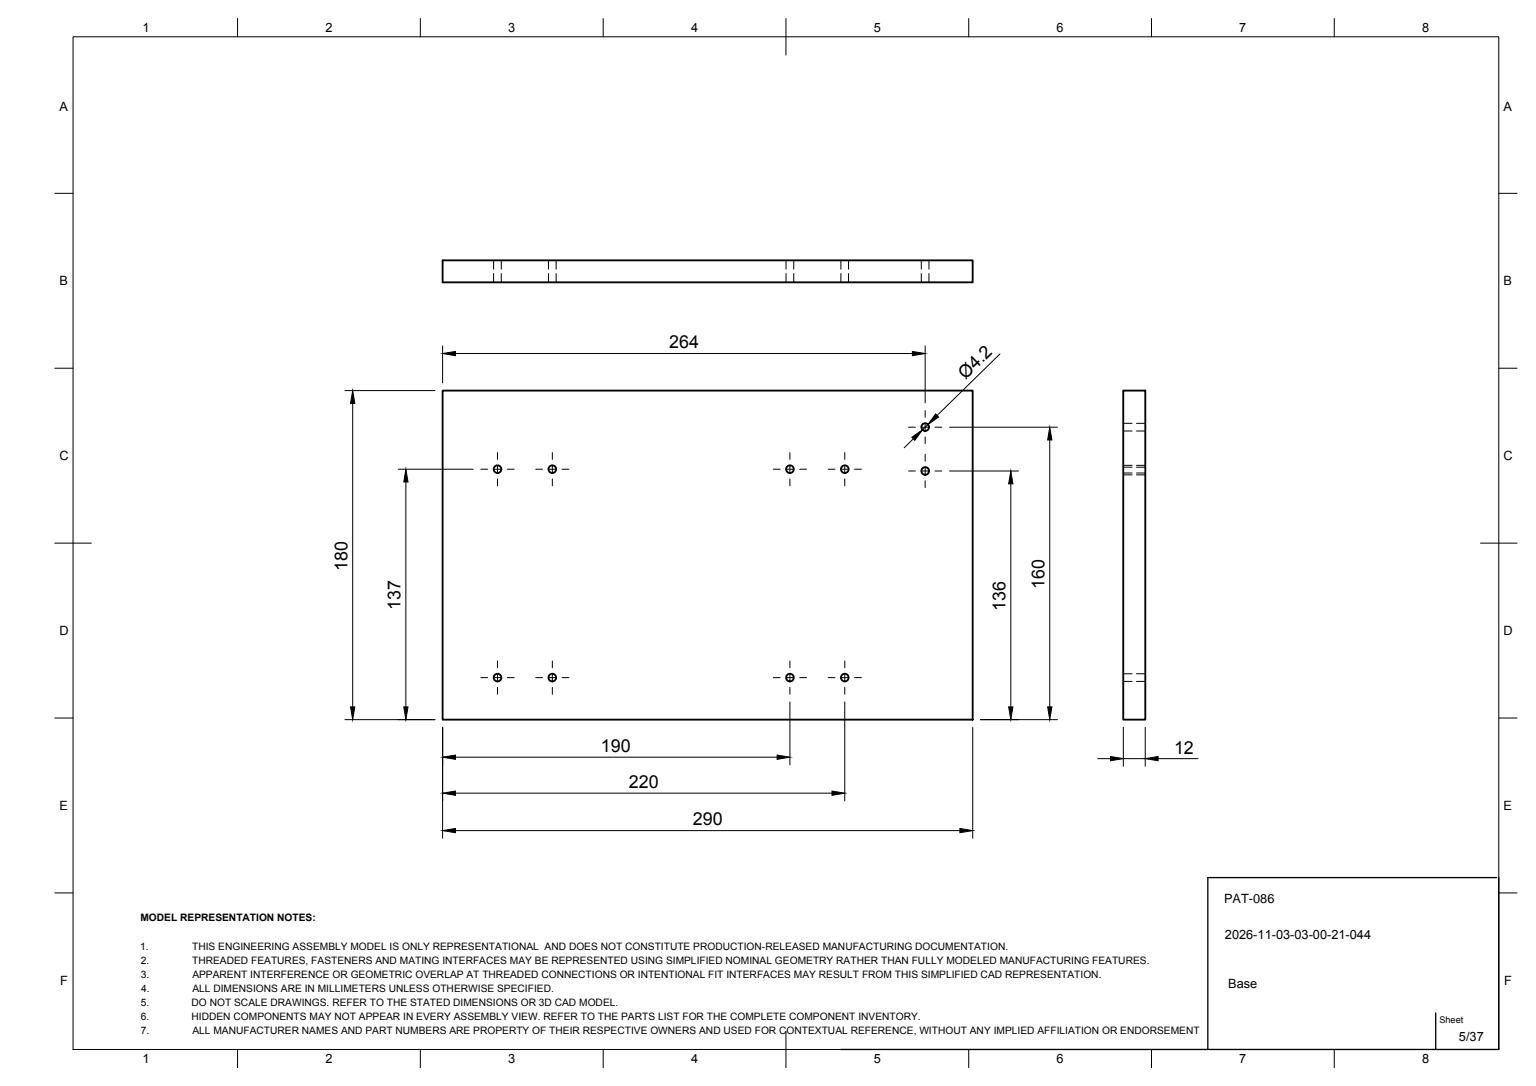
ISO-10303-21;
HEADER;
/* Generated by software containing ST-Developer
 * from STEP Tools, Inc. (www.steptools.com) 
 */

FILE_DESCRIPTION(
/* description */ ('Ratchet and pawl hand winch drum'),
/* implementation_level */ '2;1');

FILE_NAME(
/* name */ 'Base.step',
/* time_stamp */ '2026-10-27T12:42:58-07:00',
/* author */ (''),
/* organization */ (''),
/* preprocessor_version */ 'ST-DEVELOPER v20.2',
/* originating_system */ 'Autodesk Translation Framework v15.17.0.0',
/* authorisation */ '');

FILE_SCHEMA (('AUTOMOTIVE_DESIGN { 1 0 10303 214 3 1 1 }'));
ENDSEC;

DATA;
#10=MECHANICAL_DESIGN_GEOMETRIC_PRESENTATION_REPRESENTATION('',(#389),#11801);
#321=SHAPE_REPRESENTATION_RELATIONSHIP('SRR','None',#11947,#355);
#355=ADVANCED_BREP_SHAPE_REPRESENTATION('',(#424),#11764);
#389=STYLED_ITEM('',(#12192),#424);
#424=MANIFOLD_SOLID_BREP('Body1',#6266);
#456=FACE_BOUND('',#1211,.T.);
#457=FACE_BOUND('',#1212,.T.);
#458=FACE_BOUND('',#1213,.T.);
#459=FACE_BOUND('',#1214,.T.);
#460=FACE_BOUND('',#1215,.T.);
#461=FACE_BOUND('',#1216,.T.);
#462=FACE_BOUND('',#1217,.T.);
#463=FACE_BOUND('',#1218,.T.);
#464=FACE_BOUND('',#1219,.T.);
#465=FACE_BOUND('',#1220,.T.);
#466=FACE_BOUND('',#1222,.T.);
#467=FACE_BOUND('',#1223,.T.);
#468=FACE_BOUND('',#1224,.T.);
#469=FACE_BOUND('',#1225,.T.);
#470=FACE_BOUND('',#1226,.T.);
#471=FACE_BOUND('',#1227,.T.);
#472=FACE_BOUND('',#1228,.T.);
#473=FACE_BOUND('',#1229,.T.);
#474=FACE_BOUND('',#1230,.T.);
#475=FACE_BOUND('',#1231,.T.);
#601=PLANE('',#6712);
#602=PLANE('',#6713);
#603=PLANE('',#6714);
#604=PLANE('',#6715);
#605=PLANE('',#6716);
#606=PLANE('',#6717);
#840=FACE_OUTER_BOUND('',#1196,.T.);
#841=FACE_OUTER_BOUND('',#1197,.T.);
#842=FACE_OUTER_BOUND('',#1198,.T.);
#843=FACE_OUTER_BOUND('',#1199,.T.);
#844=FACE_OUTER_BOUND('',#1200,.T.);
#845=FACE_OUTER_BOUND('',#1201,.T.);
#846=FACE_OUTER_BOUND('',#1202,.T.);
#847=FACE_OUTER_BOUND('',#1203,.T.);
#848=FACE_OUTER_BOUND('',#1204,.T.);
#849=FACE_OUTER_BOUND('',#1205,.T.);
#850=FACE_OUTER_BOUND('',#1206,.T.);
#851=FACE_OUTER_BOUND('',#1207,.T.);
#852=FACE_OUTER_BOUND('',#1208,.T.);
#853=FACE_OUTER_BOUND('',#1209,.T.);
#854=FACE_OUTER_BOUND('',#1210,.T.);
#855=FACE_OUTER_BOUND('',#1221,.T.);
#1196=EDGE_LOOP('',(#4247,#4248,#4249,#4250));
#1197=EDGE_LOOP('',(#4251,#4252,#4253,#4254));
#1198=EDGE_LOOP('',(#4255,#4256,#4257,#4258));
#1199=EDGE_LOOP('',(#4259,#4260,#4261,#4262));
#1200=EDGE_LOOP('',(#4263,#4264,#4265,#4266));
#1201=EDGE_LOOP('',(#4267,#4268,#4269,#4270));
#1202=EDGE_LOOP('',(#4271,#4272,#4273,#4274));
#1203=EDGE_LOOP('',(#4275,#4276,#4277,#4278));
#1204=EDGE_LOOP('',(#4279,#4280,#4281,#4282));
#1205=EDGE_LOOP('',(#4283,#4284,#4285,#4286));
#1206=EDGE_LOOP('',(#4287,#4288,#4289,#4290));
#1207=EDGE_LOOP('',(#4291,#4292,#4293,#4294));
#1208=EDGE_LOOP('',(#4295,#4296,#4297,#4298));
#1209=EDGE_LOOP('',(#4299,#4300,#4301,#4302));
#1210=EDGE_LOOP('',(#4303,#4304,#4305,#4306));
#1211=EDGE_LOOP('',(#4307));
#1212=EDGE_LOOP('',(#4308));
#1213=EDGE_LOOP('',(#4309));
#1214=EDGE_LOOP('',(#4310));
#1215=EDGE_LOOP('',(#4311));
#1216=EDGE_LOOP('',(#4312));
#1217=EDGE_LOOP('',(#4313));
#1218=EDGE_LOOP('',(#4314));
#1219=EDGE_LOOP('',(#4315));
#1220=EDGE_LOOP('',(#4316));
#1221=EDGE_LOOP('',(#4317,#4318,#4319,#4320));
#1222=EDGE_LOOP('',(#4321));
#1223=EDGE_LOOP('',(#4322));
#1224=EDGE_LOOP('',(#4323));
#1225=EDGE_LOOP('',(#4324));
#1226=EDGE_LOOP('',(#4325));
#1227=EDGE_LOOP('',(#4326));
#1228=EDGE_LOOP('',(#4327));
#1229=EDGE_LOOP('',(#4328));
#1230=EDGE_LOOP('',(#4329));
#1231=EDGE_LOOP('',(#4330));
#1697=LINE('',#9234,#2208);
#1698=LINE('',#9240,#2209);
#1699=LINE('',#9246,#2210);
#1700=LINE('',#9252,#2211);
#1701=LINE('',#9258,#2212);
#1702=LINE('',#9264,#2213);
#1703=LINE('',#9270,#2214);
#1704=LINE('',#9276,#2215);
#1705=LINE('',#9282,#2216);
#1706=LINE('',#9288,#2217);
#1707=LINE('',#9293,#2218);
#1708=LINE('',#9295,#2219);
#1709=LINE('',#9297,#2220);
#1710=LINE('',#9298,#2221);
#1711=LINE('',#9301,#2222);
#1712=LINE('',#9303,#2223);
#1713=LINE('',#9304,#2224);
#1714=LINE('',#9307,#2225);
#1715=LINE('',#9309,#2226);
#1716=LINE('',#9310,#2227);
#1717=LINE('',#9312,#2228);
#1718=LINE('',#9313,#2229);
#2208=VECTOR('',#7368,0.210000000000001);
#2209=VECTOR('',#7375,0.21);
#2210=VECTOR('',#7382,0.21);
#2211=VECTOR('',#7389,0.21);
#2212=VECTOR('',#7396,0.21);
#2213=VECTOR('',#7403,0.21);
#2214=VECTOR('',#7410,0.21);
#2215=VECTOR('',#7417,0.21);
#2216=VECTOR('',#7424,0.21);
#2217=VECTOR('',#7431,0.21);
#2218=VECTOR('',#7436,1.);
#2219=VECTOR('',#7437,1.);
#2220=VECTOR('',#7438,1.);
#2221=VECTOR('',#7439,1.);
#2222=VECTOR('',#7442,1.);
#2223=VECTOR('',#7443,1.);
#2224=VECTOR('',#7444,1.);
#2225=VECTOR('',#7447,1.);
#2226=VECTOR('',#7448,1.);
#2227=VECTOR('',#7449,1.);
#2228=VECTOR('',#7452,1.);
#2229=VECTOR('',#7453,1.);
#2719=CIRCLE('',#6683,0.210000000000001);
#2720=CIRCLE('',#6684,0.210000000000001);
#2721=CIRCLE('',#6686,0.21);
#2722=CIRCLE('',#6687,0.21);
#2723=CIRCLE('',#6689,0.21);
#2724=CIRCLE('',#6690,0.21);
#2725=CIRCLE('',#6692,0.21);
#2726=CIRCLE('',#6693,0.21);
#2727=CIRCLE('',#6695,0.21);
#2728=CIRCLE('',#6696,0.21);
#2729=CIRCLE('',#6698,0.21);
#2730=CIRCLE('',#6699,0.21);
#2731=CIRCLE('',#6701,0.21);
#2732=CIRCLE('',#6702,0.21);
#2733=CIRCLE('',#6704,0.21);
#2734=CIRCLE('',#6705,0.21);
#2735=CIRCLE('',#6707,0.21);
#2736=CIRCLE('',#6708,0.21);
#2737=CIRCLE('',#6710,0.21);
#2738=CIRCLE('',#6711,0.21);
#2942=VERTEX_POINT('',#9231);
#2943=VERTEX_POINT('',#9233);
#2944=VERTEX_POINT('',#9237);
#2945=VERTEX_POINT('',#9239);
#2946=VERTEX_POINT('',#9243);
#2947=VERTEX_POINT('',#9245);
#2948=VERTEX_POINT('',#9249);
#2949=VERTEX_POINT('',#9251);
#2950=VERTEX_POINT('',#9255);
#2951=VERTEX_POINT('',#9257);
#2952=VERTEX_POINT('',#9261);
#2953=VERTEX_POINT('',#9263);
#2954=VERTEX_POINT('',#9267);
#2955=VERTEX_POINT('',#9269);
#2956=VERTEX_POINT('',#9273);
#2957=VERTEX_POINT('',#9275);
#2958=VERTEX_POINT('',#9279);
#2959=VERTEX_POINT('',#9281);
#2960=VERTEX_POINT('',#9285);
#2961=VERTEX_POINT('',#9287);
#2962=VERTEX_POINT('',#9291);
#2963=VERTEX_POINT('',#9292);
#2964=VERTEX_POINT('',#9294);
#2965=VERTEX_POINT('',#9296);
#2966=VERTEX_POINT('',#9300);
#2967=VERTEX_POINT('',#9302);
#2968=VERTEX_POINT('',#9306);
#2969=VERTEX_POINT('',#9308);
#3467=EDGE_CURVE('',#2942,#2942,#2719,.T.);
#3468=EDGE_CURVE('',#2942,#2943,#1697,.T.);
#3469=EDGE_CURVE('',#2943,#2943,#2720,.T.);
#3470=EDGE_CURVE('',#2944,#2944,#2721,.T.);
#3471=EDGE_CURVE('',#2944,#2945,#1698,.T.);
#3472=EDGE_CURVE('',#2945,#2945,#2722,.T.);
#3473=EDGE_CURVE('',#2946,#2946,#2723,.T.);
#3474=EDGE_CURVE('',#2946,#2947,#1699,.T.);
#3475=EDGE_CURVE('',#2947,#2947,#2724,.T.);
#3476=EDGE_CURVE('',#2948,#2948,#2725,.T.);
#3477=EDGE_CURVE('',#2948,#2949,#1700,.T.);
#3478=EDGE_CURVE('',#2949,#2949,#2726,.T.);
#3479=EDGE_CURVE('',#2950,#2950,#2727,.T.);
#3480=EDGE_CURVE('',#2950,#2951,#1701,.T.);
#3481=EDGE_CURVE('',#2951,#2951,#2728,.T.);
#3482=EDGE_CURVE('',#2952,#2952,#2729,.T.);
#3483=EDGE_CURVE('',#2952,#2953,#1702,.T.);
#3484=EDGE_CURVE('',#2953,#2953,#2730,.T.);
#3485=EDGE_CURVE('',#2954,#2954,#2731,.T.);
#3486=EDGE_CURVE('',#2954,#2955,#1703,.T.);
#3487=EDGE_CURVE('',#2955,#2955,#2732,.T.);
#3488=EDGE_CURVE('',#2956,#2956,#2733,.T.);
#3489=EDGE_CURVE('',#2956,#2957,#1704,.T.);
#3490=EDGE_CURVE('',#2957,#2957,#2734,.T.);
#3491=EDGE_CURVE('',#2958,#2958,#2735,.T.);
#3492=EDGE_CURVE('',#2958,#2959,#1705,.T.);
#3493=EDGE_CURVE('',#2959,#2959,#2736,.T.);
#3494=EDGE_CURVE('',#2960,#2960,#2737,.T.);
#3495=EDGE_CURVE('',#2960,#2961,#1706,.T.);
#3496=EDGE_CURVE('',#2961,#2961,#2738,.T.);
#3497=EDGE_CURVE('',#2962,#2963,#1707,.T.);
#3498=EDGE_CURVE('',#2963,#2964,#1708,.T.);
#3499=EDGE_CURVE('',#2965,#2964,#1709,.T.);
#3500=EDGE_CURVE('',#2962,#2965,#1710,.T.);
#3501=EDGE_CURVE('',#2966,#2962,#1711,.T.);
#3502=EDGE_CURVE('',#2967,#2965,#1712,.T.);
#3503=EDGE_CURVE('',#2966,#2967,#1713,.T.);
#3504=EDGE_CURVE('',#2968,#2966,#1714,.T.);
#3505=EDGE_CURVE('',#2969,#2967,#1715,.T.);
#3506=EDGE_CURVE('',#2968,#2969,#1716,.T.);
#3507=EDGE_CURVE('',#2963,#2968,#1717,.T.);
#3508=EDGE_CURVE('',#2964,#2969,#1718,.T.);
#4247=ORIENTED_EDGE('',*,*,#3467,.F.);
#4248=ORIENTED_EDGE('',*,*,#3468,.T.);
#4249=ORIENTED_EDGE('',*,*,#3469,.F.);
#4250=ORIENTED_EDGE('',*,*,#3468,.F.);
#4251=ORIENTED_EDGE('',*,*,#3470,.F.);
#4252=ORIENTED_EDGE('',*,*,#3471,.T.);
#4253=ORIENTED_EDGE('',*,*,#3472,.F.);
#4254=ORIENTED_EDGE('',*,*,#3471,.F.);
#4255=ORIENTED_EDGE('',*,*,#3473,.F.);
#4256=ORIENTED_EDGE('',*,*,#3474,.T.);
#4257=ORIENTED_EDGE('',*,*,#3475,.F.);
#4258=ORIENTED_EDGE('',*,*,#3474,.F.);
#4259=ORIENTED_EDGE('',*,*,#3476,.F.);
#4260=ORIENTED_EDGE('',*,*,#3477,.T.);
#4261=ORIENTED_EDGE('',*,*,#3478,.F.);
#4262=ORIENTED_EDGE('',*,*,#3477,.F.);
#4263=ORIENTED_EDGE('',*,*,#3479,.F.);
#4264=ORIENTED_EDGE('',*,*,#3480,.T.);
#4265=ORIENTED_EDGE('',*,*,#3481,.F.);
#4266=ORIENTED_EDGE('',*,*,#3480,.F.);
#4267=ORIENTED_EDGE('',*,*,#3482,.F.);
#4268=ORIENTED_EDGE('',*,*,#3483,.T.);
#4269=ORIENTED_EDGE('',*,*,#3484,.F.);
#4270=ORIENTED_EDGE('',*,*,#3483,.F.);
#4271=ORIENTED_EDGE('',*,*,#3485,.F.);
#4272=ORIENTED_EDGE('',*,*,#3486,.T.);
#4273=ORIENTED_EDGE('',*,*,#3487,.F.);
#4274=ORIENTED_EDGE('',*,*,#3486,.F.);
#4275=ORIENTED_EDGE('',*,*,#3488,.F.);
#4276=ORIENTED_EDGE('',*,*,#3489,.T.);
#4277=ORIENTED_EDGE('',*,*,#3490,.F.);
#4278=ORIENTED_EDGE('',*,*,#3489,.F.);
#4279=ORIENTED_EDGE('',*,*,#3491,.F.);
#4280=ORIENTED_EDGE('',*,*,#3492,.T.);
#4281=ORIENTED_EDGE('',*,*,#3493,.F.);
#4282=ORIENTED_EDGE('',*,*,#3492,.F.);
#4283=ORIENTED_EDGE('',*,*,#3494,.F.);
#4284=ORIENTED_EDGE('',*,*,#3495,.T.);
#4285=ORIENTED_EDGE('',*,*,#3496,.F.);
#4286=ORIENTED_EDGE('',*,*,#3495,.F.);
#4287=ORIENTED_EDGE('',*,*,#3497,.T.);
#4288=ORIENTED_EDGE('',*,*,#3498,.T.);
#4289=ORIENTED_EDGE('',*,*,#3499,.F.);
#4290=ORIENTED_EDGE('',*,*,#3500,.F.);
#4291=ORIENTED_EDGE('',*,*,#3501,.T.);
#4292=ORIENTED_EDGE('',*,*,#3500,.T.);
#4293=ORIENTED_EDGE('',*,*,#3502,.F.);
#4294=ORIENTED_EDGE('',*,*,#3503,.F.);
#4295=ORIENTED_EDGE('',*,*,#3504,.T.);
#4296=ORIENTED_EDGE('',*,*,#3503,.T.);
#4297=ORIENTED_EDGE('',*,*,#3505,.F.);
#4298=ORIENTED_EDGE('',*,*,#3506,.F.);
#4299=ORIENTED_EDGE('',*,*,#3507,.T.);
#4300=ORIENTED_EDGE('',*,*,#3506,.T.);
#4301=ORIENTED_EDGE('',*,*,#3508,.F.);
#4302=ORIENTED_EDGE('',*,*,#3498,.F.);
#4303=ORIENTED_EDGE('',*,*,#3508,.T.);
#4304=ORIENTED_EDGE('',*,*,#3505,.T.);
#4305=ORIENTED_EDGE('',*,*,#3502,.T.);
#4306=ORIENTED_EDGE('',*,*,#3499,.T.);
#4307=ORIENTED_EDGE('',*,*,#3472,.T.);
#4308=ORIENTED_EDGE('',*,*,#3496,.T.);
#4309=ORIENTED_EDGE('',*,*,#3493,.T.);
#4310=ORIENTED_EDGE('',*,*,#3490,.T.);
#4311=ORIENTED_EDGE('',*,*,#3487,.T.);
#4312=ORIENTED_EDGE('',*,*,#3484,.T.);
#4313=ORIENTED_EDGE('',*,*,#3481,.T.);
#4314=ORIENTED_EDGE('',*,*,#3478,.T.);
#4315=ORIENTED_EDGE('',*,*,#3475,.T.);
#4316=ORIENTED_EDGE('',*,*,#3469,.T.);
#4317=ORIENTED_EDGE('',*,*,#3507,.F.);
#4318=ORIENTED_EDGE('',*,*,#3497,.F.);
#4319=ORIENTED_EDGE('',*,*,#3501,.F.);
#4320=ORIENTED_EDGE('',*,*,#3504,.F.);
#4321=ORIENTED_EDGE('',*,*,#3470,.T.);
#4322=ORIENTED_EDGE('',*,*,#3494,.T.);
#4323=ORIENTED_EDGE('',*,*,#3491,.T.);
#4324=ORIENTED_EDGE('',*,*,#3488,.T.);
#4325=ORIENTED_EDGE('',*,*,#3485,.T.);
#4326=ORIENTED_EDGE('',*,*,#3482,.T.);
#4327=ORIENTED_EDGE('',*,*,#3479,.T.);
#4328=ORIENTED_EDGE('',*,*,#3476,.T.);
#4329=ORIENTED_EDGE('',*,*,#3473,.T.);
#4330=ORIENTED_EDGE('',*,*,#3467,.T.);
#5807=CYLINDRICAL_SURFACE('',#6682,0.210000000000001);
#5808=CYLINDRICAL_SURFACE('',#6685,0.21);
#5809=CYLINDRICAL_SURFACE('',#6688,0.21);
#5810=CYLINDRICAL_SURFACE('',#6691,0.21);
#5811=CYLINDRICAL_SURFACE('',#6694,0.21);
#5812=CYLINDRICAL_SURFACE('',#6697,0.21);
#5813=CYLINDRICAL_SURFACE('',#6700,0.21);
#5814=CYLINDRICAL_SURFACE('',#6703,0.21);
#5815=CYLINDRICAL_SURFACE('',#6706,0.21);
#5816=CYLINDRICAL_SURFACE('',#6709,0.21);
#5910=ADVANCED_FACE('',(#840),#5807,.F.);
#5911=ADVANCED_FACE('',(#841),#5808,.F.);
#5912=ADVANCED_FACE('',(#842),#5809,.F.);
#5913=ADVANCED_FACE('',(#843),#5810,.F.);
#5914=ADVANCED_FACE('',(#844),#5811,.F.);
#5915=ADVANCED_FACE('',(#845),#5812,.F.);
#5916=ADVANCED_FACE('',(#846),#5813,.F.);
#5917=ADVANCED_FACE('',(#847),#5814,.F.);
#5918=ADVANCED_FACE('',(#848),#5815,.F.);
#5919=ADVANCED_FACE('',(#849),#5816,.F.);
#5920=ADVANCED_FACE('',(#850),#601,.T.);
#5921=ADVANCED_FACE('',(#851),#602,.T.);
#5922=ADVANCED_FACE('',(#852),#603,.T.);
#5923=ADVANCED_FACE('',(#853),#604,.T.);
#5924=ADVANCED_FACE('',(#854,#456,#457,#458,#459,#460,#461,#462,#463,#464,
#465),#605,.T.);
#5925=ADVANCED_FACE('',(#855,#466,#467,#468,#469,#470,#471,#472,#473,#474,
#475),#606,.F.);
#6266=CLOSED_SHELL('',(#5910,#5911,#5912,#5913,#5914,#5915,#5916,#5917,
#5918,#5919,#5920,#5921,#5922,#5923,#5924,#5925));
#6681=AXIS2_PLACEMENT_3D('',#9229,#7362,#7363);
#6682=AXIS2_PLACEMENT_3D('',#9230,#7364,#7365);
#6683=AXIS2_PLACEMENT_3D('',#9232,#7366,#7367);
#6684=AXIS2_PLACEMENT_3D('',#9235,#7369,#7370);
#6685=AXIS2_PLACEMENT_3D('',#9236,#7371,#7372);
#6686=AXIS2_PLACEMENT_3D('',#9238,#7373,#7374);
#6687=AXIS2_PLACEMENT_3D('',#9241,#7376,#7377);
#6688=AXIS2_PLACEMENT_3D('',#9242,#7378,#7379);
#6689=AXIS2_PLACEMENT_3D('',#9244,#7380,#7381);
#6690=AXIS2_PLACEMENT_3D('',#9247,#7383,#7384);
#6691=AXIS2_PLACEMENT_3D('',#9248,#7385,#7386);
#6692=AXIS2_PLACEMENT_3D('',#9250,#7387,#7388);
#6693=AXIS2_PLACEMENT_3D('',#9253,#7390,#7391);
#6694=AXIS2_PLACEMENT_3D('',#9254,#7392,#7393);
#6695=AXIS2_PLACEMENT_3D('',#9256,#7394,#7395);
#6696=AXIS2_PLACEMENT_3D('',#9259,#7397,#7398);
#6697=AXIS2_PLACEMENT_3D('',#9260,#7399,#7400);
#6698=AXIS2_PLACEMENT_3D('',#9262,#7401,#7402);
#6699=AXIS2_PLACEMENT_3D('',#9265,#7404,#7405);
#6700=AXIS2_PLACEMENT_3D('',#9266,#7406,#7407);
#6701=AXIS2_PLACEMENT_3D('',#9268,#7408,#7409);
#6702=AXIS2_PLACEMENT_3D('',#9271,#7411,#7412);
#6703=AXIS2_PLACEMENT_3D('',#9272,#7413,#7414);
#6704=AXIS2_PLACEMENT_3D('',#9274,#7415,#7416);
#6705=AXIS2_PLACEMENT_3D('',#9277,#7418,#7419);
#6706=AXIS2_PLACEMENT_3D('',#9278,#7420,#7421);
#6707=AXIS2_PLACEMENT_3D('',#9280,#7422,#7423);
#6708=AXIS2_PLACEMENT_3D('',#9283,#7425,#7426);
#6709=AXIS2_PLACEMENT_3D('',#9284,#7427,#7428);
#6710=AXIS2_PLACEMENT_3D('',#9286,#7429,#7430);
#6711=AXIS2_PLACEMENT_3D('',#9289,#7432,#7433);
#6712=AXIS2_PLACEMENT_3D('',#9290,#7434,#7435);
#6713=AXIS2_PLACEMENT_3D('',#9299,#7440,#7441);
#6714=AXIS2_PLACEMENT_3D('',#9305,#7445,#7446);
#6715=AXIS2_PLACEMENT_3D('',#9311,#7450,#7451);
#6716=AXIS2_PLACEMENT_3D('',#9314,#7454,#7455);
#6717=AXIS2_PLACEMENT_3D('',#9315,#7456,#7457);
#7362=DIRECTION('axis',(0.,0.,1.));
#7363=DIRECTION('refdir',(1.,0.,0.));
#7364=DIRECTION('center_axis',(0.,0.,1.));
#7365=DIRECTION('ref_axis',(1.,0.,0.));
#7366=DIRECTION('center_axis',(0.,0.,1.));
#7367=DIRECTION('ref_axis',(1.,0.,0.));
#7368=DIRECTION('',(0.,0.,1.));
#7369=DIRECTION('center_axis',(0.,0.,-1.));
#7370=DIRECTION('ref_axis',(1.,0.,0.));
#7371=DIRECTION('center_axis',(0.,0.,1.));
#7372=DIRECTION('ref_axis',(1.,0.,0.));
#7373=DIRECTION('center_axis',(0.,0.,1.));
#7374=DIRECTION('ref_axis',(1.,0.,0.));
#7375=DIRECTION('',(0.,0.,1.));
#7376=DIRECTION('center_axis',(0.,0.,-1.));
#7377=DIRECTION('ref_axis',(1.,0.,0.));
#7378=DIRECTION('center_axis',(0.,0.,1.));
#7379=DIRECTION('ref_axis',(1.,0.,0.));
#7380=DIRECTION('center_axis',(0.,0.,1.));
#7381=DIRECTION('ref_axis',(1.,0.,0.));
#7382=DIRECTION('',(0.,0.,1.));
#7383=DIRECTION('center_axis',(0.,0.,-1.));
#7384=DIRECTION('ref_axis',(1.,0.,0.));
#7385=DIRECTION('center_axis',(0.,0.,1.));
#7386=DIRECTION('ref_axis',(1.,0.,0.));
#7387=DIRECTION('center_axis',(0.,0.,1.));
#7388=DIRECTION('ref_axis',(1.,0.,0.));
#7389=DIRECTION('',(0.,0.,1.));
#7390=DIRECTION('center_axis',(0.,0.,-1.));
#7391=DIRECTION('ref_axis',(1.,0.,0.));
#7392=DIRECTION('center_axis',(0.,0.,1.));
#7393=DIRECTION('ref_axis',(1.,0.,0.));
#7394=DIRECTION('center_axis',(0.,0.,1.));
#7395=DIRECTION('ref_axis',(1.,0.,0.));
#7396=DIRECTION('',(0.,0.,1.));
#7397=DIRECTION('center_axis',(0.,0.,-1.));
#7398=DIRECTION('ref_axis',(1.,0.,0.));
#7399=DIRECTION('center_axis',(0.,0.,1.));
#7400=DIRECTION('ref_axis',(1.,0.,0.));
#7401=DIRECTION('center_axis',(0.,0.,1.));
#7402=DIRECTION('ref_axis',(1.,0.,0.));
#7403=DIRECTION('',(0.,0.,1.));
#7404=DIRECTION('center_axis',(0.,0.,-1.));
#7405=DIRECTION('ref_axis',(1.,0.,0.));
#7406=DIRECTION('center_axis',(0.,0.,1.));
#7407=DIRECTION('ref_axis',(1.,0.,0.));
#7408=DIRECTION('center_axis',(0.,0.,1.));
#7409=DIRECTION('ref_axis',(1.,0.,0.));
#7410=DIRECTION('',(0.,0.,1.));
#7411=DIRECTION('center_axis',(0.,0.,-1.));
#7412=DIRECTION('ref_axis',(1.,0.,0.));
#7413=DIRECTION('center_axis',(0.,0.,1.));
#7414=DIRECTION('ref_axis',(1.,0.,0.));
#7415=DIRECTION('center_axis',(0.,0.,1.));
#7416=DIRECTION('ref_axis',(1.,0.,0.));
#7417=DIRECTION('',(0.,0.,1.));
#7418=DIRECTION('center_axis',(0.,0.,-1.));
#7419=DIRECTION('ref_axis',(1.,0.,0.));
#7420=DIRECTION('center_axis',(0.,0.,1.));
#7421=DIRECTION('ref_axis',(1.,0.,0.));
#7422=DIRECTION('center_axis',(0.,0.,1.));
#7423=DIRECTION('ref_axis',(1.,0.,0.));
#7424=DIRECTION('',(0.,0.,1.));
#7425=DIRECTION('center_axis',(0.,0.,-1.));
#7426=DIRECTION('ref_axis',(1.,0.,0.));
#7427=DIRECTION('center_axis',(0.,0.,1.));
#7428=DIRECTION('ref_axis',(1.,0.,0.));
#7429=DIRECTION('center_axis',(0.,0.,1.));
#7430=DIRECTION('ref_axis',(1.,0.,0.));
#7431=DIRECTION('',(0.,0.,1.));
#7432=DIRECTION('center_axis',(0.,0.,-1.));
#7433=DIRECTION('ref_axis',(1.,0.,0.));
#7434=DIRECTION('center_axis',(0.,1.,0.));
#7435=DIRECTION('ref_axis',(-1.,0.,0.));
#7436=DIRECTION('',(-1.,0.,0.));
#7437=DIRECTION('',(0.,0.,1.));
#7438=DIRECTION('',(-1.,0.,0.));
#7439=DIRECTION('',(0.,0.,1.));
#7440=DIRECTION('center_axis',(1.,0.,0.));
#7441=DIRECTION('ref_axis',(0.,1.,0.));
#7442=DIRECTION('',(0.,1.,0.));
#7443=DIRECTION('',(0.,1.,0.));
#7444=DIRECTION('',(0.,0.,1.));
#7445=DIRECTION('center_axis',(0.,-1.,0.));
#7446=DIRECTION('ref_axis',(1.,0.,0.));
#7447=DIRECTION('',(1.,0.,0.));
#7448=DIRECTION('',(1.,0.,0.));
#7449=DIRECTION('',(0.,0.,1.));
#7450=DIRECTION('center_axis',(-1.,0.,0.));
#7451=DIRECTION('ref_axis',(0.,-1.,0.));
#7452=DIRECTION('',(0.,-1.,0.));
#7453=DIRECTION('',(0.,-1.,0.));
#7454=DIRECTION('center_axis',(0.,0.,1.));
#7455=DIRECTION('ref_axis',(1.,0.,0.));
#7456=DIRECTION('center_axis',(0.,0.,1.));
#7457=DIRECTION('ref_axis',(1.,0.,0.));
#9229=CARTESIAN_POINT('',(0.,0.,0.));
#9230=CARTESIAN_POINT('Origin',(8.,-5.9,-0.1));
#9231=CARTESIAN_POINT('',(7.79,-5.9,0.));
#9232=CARTESIAN_POINT('Origin',(8.,-5.9,0.));
#9233=CARTESIAN_POINT('',(7.79,-5.9,1.2));
#9234=CARTESIAN_POINT('',(7.79,-5.9,-0.1));
#9235=CARTESIAN_POINT('Origin',(8.,-5.9,1.2));
#9236=CARTESIAN_POINT('Origin',(5.6,-5.9,-0.1));
#9237=CARTESIAN_POINT('',(5.39,-5.9,0.));
#9238=CARTESIAN_POINT('Origin',(5.6,-5.9,0.));
#9239=CARTESIAN_POINT('',(5.39,-5.9,1.2));
#9240=CARTESIAN_POINT('',(5.39,-5.9,-0.1));
#9241=CARTESIAN_POINT('Origin',(5.6,-5.9,1.2));
#9242=CARTESIAN_POINT('Origin',(5.7,14.5,-0.1));
#9243=CARTESIAN_POINT('',(5.49,14.5,0.));
#9244=CARTESIAN_POINT('Origin',(5.7,14.5,0.));
#9245=CARTESIAN_POINT('',(5.49,14.5,1.2));
#9246=CARTESIAN_POINT('',(5.49,14.5,-0.1));
#9247=CARTESIAN_POINT('Origin',(5.7,14.5,1.2));
#9248=CARTESIAN_POINT('Origin',(5.7,17.5,-0.1));
#9249=CARTESIAN_POINT('',(5.49,17.5,0.));
#9250=CARTESIAN_POINT('Origin',(5.7,17.5,0.));
#9251=CARTESIAN_POINT('',(5.49,17.5,1.2));
#9252=CARTESIAN_POINT('',(5.49,17.5,-0.1));
#9253=CARTESIAN_POINT('Origin',(5.7,17.5,1.2));
#9254=CARTESIAN_POINT('Origin',(-5.7,14.5,-0.1));
#9255=CARTESIAN_POINT('',(-5.91,14.5,0.));
#9256=CARTESIAN_POINT('Origin',(-5.7,14.5,0.));
#9257=CARTESIAN_POINT('',(-5.91,14.5,1.2));
#9258=CARTESIAN_POINT('',(-5.91,14.5,-0.1));
#9259=CARTESIAN_POINT('Origin',(-5.7,14.5,1.2));
#9260=CARTESIAN_POINT('Origin',(-5.7,17.5,-0.1));
#9261=CARTESIAN_POINT('',(-5.91,17.5,0.));
#9262=CARTESIAN_POINT('Origin',(-5.7,17.5,0.));
#9263=CARTESIAN_POINT('',(-5.91,17.5,1.2));
#9264=CARTESIAN_POINT('',(-5.91,17.5,-0.1));
#9265=CARTESIAN_POINT('Origin',(-5.7,17.5,1.2));
#9266=CARTESIAN_POINT('Origin',(5.7,-1.5,-0.1));
#9267=CARTESIAN_POINT('',(5.49,-1.5,0.));
#9268=CARTESIAN_POINT('Origin',(5.7,-1.5,0.));
#9269=CARTESIAN_POINT('',(5.49,-1.5,1.2));
#9270=CARTESIAN_POINT('',(5.49,-1.5,-0.1));
#9271=CARTESIAN_POINT('Origin',(5.7,-1.5,1.2));
#9272=CARTESIAN_POINT('Origin',(5.7,1.5,-0.1));
#9273=CARTESIAN_POINT('',(5.49,1.5,0.));
#9274=CARTESIAN_POINT('Origin',(5.7,1.5,0.));
#9275=CARTESIAN_POINT('',(5.49,1.5,1.2));
#9276=CARTESIAN_POINT('',(5.49,1.5,-0.1));
#9277=CARTESIAN_POINT('Origin',(5.7,1.5,1.2));
#9278=CARTESIAN_POINT('Origin',(-5.7,-1.5,-0.1));
#9279=CARTESIAN_POINT('',(-5.91,-1.5,0.));
#9280=CARTESIAN_POINT('Origin',(-5.7,-1.5,0.));
#9281=CARTESIAN_POINT('',(-5.91,-1.5,1.2));
#9282=CARTESIAN_POINT('',(-5.91,-1.5,-0.1));
#9283=CARTESIAN_POINT('Origin',(-5.7,-1.5,1.2));
#9284=CARTESIAN_POINT('Origin',(-5.7,1.5,-0.1));
#9285=CARTESIAN_POINT('',(-5.91,1.5,0.));
#9286=CARTESIAN_POINT('Origin',(-5.7,1.5,0.));
#9287=CARTESIAN_POINT('',(-5.91,1.5,1.2));
#9288=CARTESIAN_POINT('',(-5.91,1.5,-0.1));
#9289=CARTESIAN_POINT('Origin',(-5.7,1.5,1.2));
#9290=CARTESIAN_POINT('Origin',(10.,20.5,0.));
#9291=CARTESIAN_POINT('',(10.,20.5,0.));
#9292=CARTESIAN_POINT('',(-8.,20.5,0.));
#9293=CARTESIAN_POINT('',(10.,20.5,0.));
#9294=CARTESIAN_POINT('',(-8.,20.5,1.2));
#9295=CARTESIAN_POINT('',(-8.,20.5,0.));
#9296=CARTESIAN_POINT('',(10.,20.5,1.2));
#9297=CARTESIAN_POINT('',(10.,20.5,1.2));
#9298=CARTESIAN_POINT('',(10.,20.5,0.));
#9299=CARTESIAN_POINT('Origin',(10.,-8.5,0.));
#9300=CARTESIAN_POINT('',(10.,-8.5,0.));
#9301=CARTESIAN_POINT('',(10.,-8.5,0.));
#9302=CARTESIAN_POINT('',(10.,-8.5,1.2));
#9303=CARTESIAN_POINT('',(10.,-8.5,1.2));
#9304=CARTESIAN_POINT('',(10.,-8.5,0.));
#9305=CARTESIAN_POINT('Origin',(-8.,-8.5,0.));
#9306=CARTESIAN_POINT('',(-8.,-8.5,0.));
#9307=CARTESIAN_POINT('',(-8.,-8.5,0.));
#9308=CARTESIAN_POINT('',(-8.,-8.5,1.2));
#9309=CARTESIAN_POINT('',(-8.,-8.5,1.2));
#9310=CARTESIAN_POINT('',(-8.,-8.5,0.));
#9311=CARTESIAN_POINT('Origin',(-8.,20.5,0.));
#9312=CARTESIAN_POINT('',(-8.,20.5,0.));
#9313=CARTESIAN_POINT('',(-8.,20.5,1.2));
#9314=CARTESIAN_POINT('Origin',(1.,6.,1.2));
#9315=CARTESIAN_POINT('Origin',(1.,6.,0.));
#11724=UNCERTAINTY_MEASURE_WITH_UNIT(LENGTH_MEASURE(0.001),#11802,
'DISTANCE_ACCURACY_VALUE',
'Maximum model space distance between geometric entities at asserted c
onnectivities');
#11761=UNCERTAINTY_MEASURE_WITH_UNIT(LENGTH_MEASURE(0.001),#11802,
'DISTANCE_ACCURACY_VALUE',
'Maximum model space distance between geometric entities at asserted c
onnectivities');
#11764=(
GEOMETRIC_REPRESENTATION_CONTEXT(3)
GLOBAL_UNCERTAINTY_ASSIGNED_CONTEXT((#11724))
GLOBAL_UNIT_ASSIGNED_CONTEXT((#11802,#11804,#11805))
REPRESENTATION_CONTEXT('','3D')
);
#11801=(
GEOMETRIC_REPRESENTATION_CONTEXT(3)
GLOBAL_UNCERTAINTY_ASSIGNED_CONTEXT((#11761))
GLOBAL_UNIT_ASSIGNED_CONTEXT((#11802,#11804,#11805))
REPRESENTATION_CONTEXT('','3D')
);
#11802=(
LENGTH_UNIT()
NAMED_UNIT(*)
SI_UNIT(.CENTI.,.METRE.)
);
#11804=(
NAMED_UNIT(*)
PLANE_ANGLE_UNIT()
SI_UNIT($,.RADIAN.)
);
#11805=(
NAMED_UNIT(*)
SI_UNIT($,.STERADIAN.)
SOLID_ANGLE_UNIT()
);
#11808=SHAPE_DEFINITION_REPRESENTATION(#11847,#11947);
#11847=PRODUCT_DEFINITION_SHAPE('',$,#11987);
#11947=SHAPE_REPRESENTATION('',(#6681),#11764);
#11984=PRODUCT_DEFINITION_CONTEXT('part definition',#12103,'design');
#11987=PRODUCT_DEFINITION('Base','Base',#12026,#11984);
#12026=PRODUCT_DEFINITION_FORMATION('',$,#12107);
#12103=APPLICATION_CONTEXT(
'Core Data for Automotive Mechanical Design Process');
#12104=PRODUCT_CONTEXT('part definition',#12103,'mechanical');
#12107=PRODUCT('Base','Base','Base',(#12104));
#12186=COLOUR_RGB('Dark Blue',0.08,0.2,0.34);
#12187=FILL_AREA_STYLE_COLOUR('',#12186);
#12188=FILL_AREA_STYLE('',(#12187));
#12189=SURFACE_STYLE_FILL_AREA(#12188);
#12190=SURFACE_SIDE_STYLE('',(#12189));
#12191=SURFACE_STYLE_USAGE(.BOTH.,#12190);
#12192=PRESENTATION_STYLE_ASSIGNMENT((#12191));
ENDSEC;
END-ISO-10303-21;
